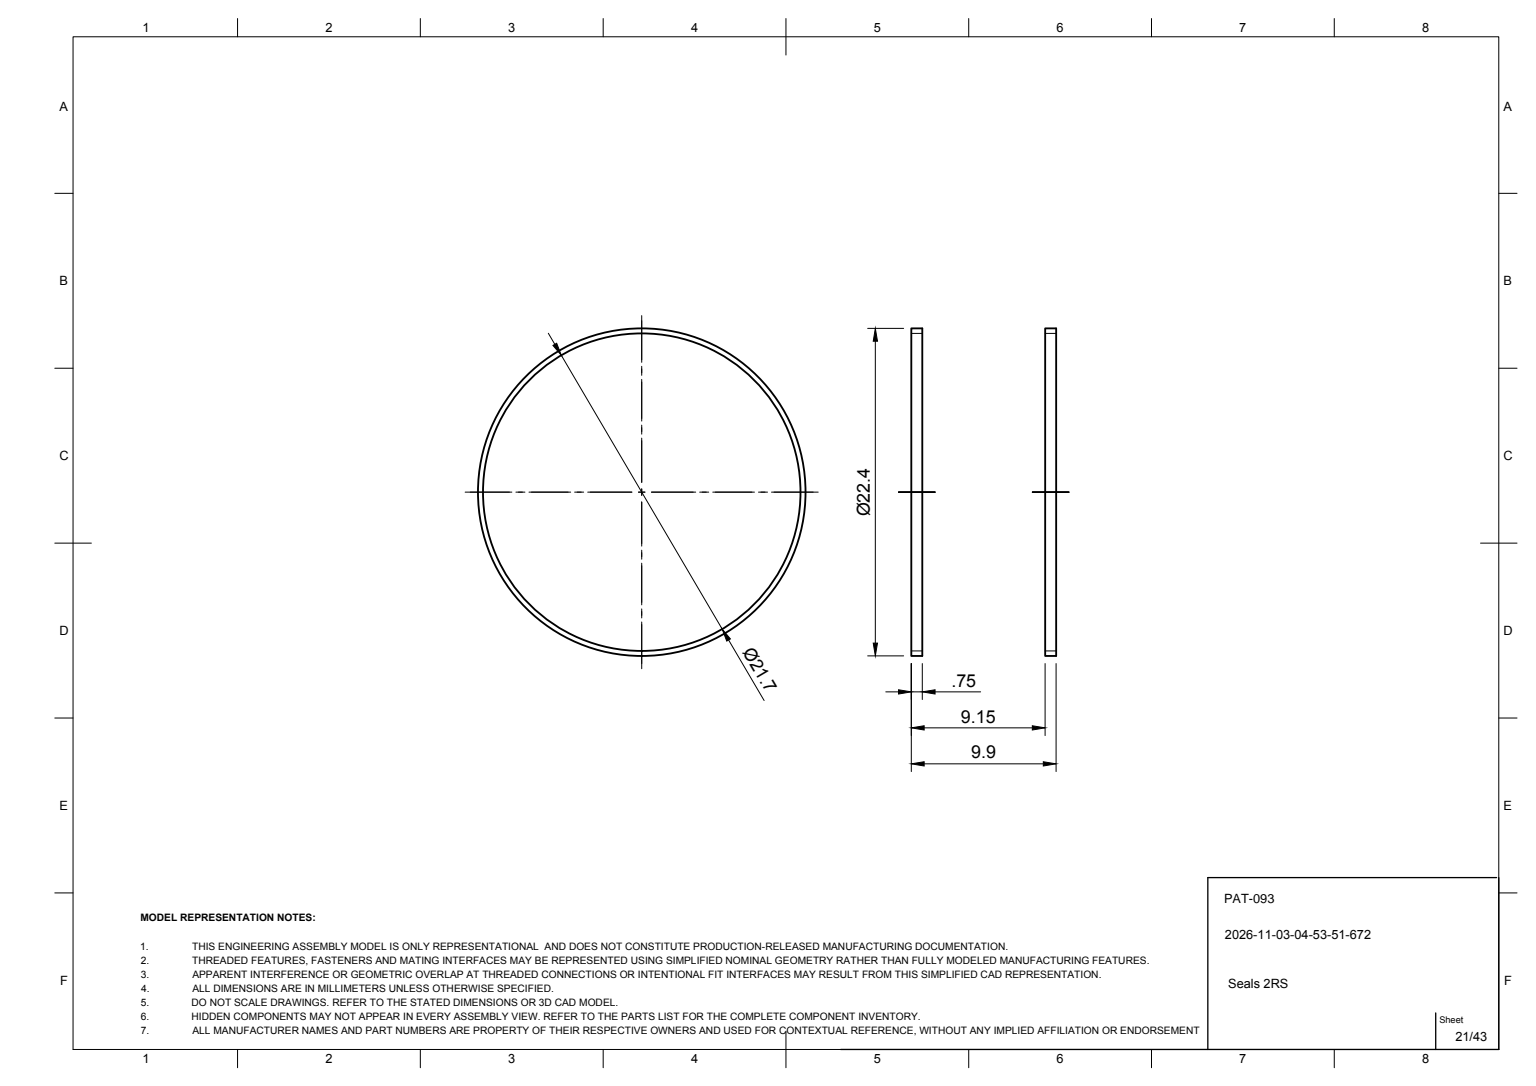
ISO-10303-21;
HEADER;
/* Generated by software containing ST-Developer
 * from STEP Tools, Inc. (www.steptools.com) 
 */

FILE_DESCRIPTION(
/* description */ ('Self-centering screw clamp'),
/* implementation_level */ '2;1');

FILE_NAME(
/* name */ 'Seals 2RS.step',
/* time_stamp */ '2026-10-28T03:25:31-07:00',
/* author */ (''),
/* organization */ (''),
/* preprocessor_version */ 'ST-DEVELOPER v20.2',
/* originating_system */ 'Autodesk Translation Framework v15.17.0.0',
/* authorisation */ '');

FILE_SCHEMA (('AUTOMOTIVE_DESIGN { 1 0 10303 214 3 1 1 }'));
ENDSEC;

DATA;
#10=MECHANICAL_DESIGN_GEOMETRIC_PRESENTATION_REPRESENTATION('',(#648,#649),#16799);
#560=SHAPE_REPRESENTATION_RELATIONSHIP('SRR','None',#17034,#601);
#601=ADVANCED_BREP_SHAPE_REPRESENTATION('',(#696,#697),#16772);
#648=STYLED_ITEM('',(#17326),#696);
#649=STYLED_ITEM('',(#17326),#697);
#696=MANIFOLD_SOLID_BREP('Body1',#9099);
#697=MANIFOLD_SOLID_BREP('Body2',#9100);
#847=FACE_BOUND('',#2128,.T.);
#848=FACE_BOUND('',#2131,.T.);
#849=FACE_BOUND('',#2134,.T.);
#850=FACE_BOUND('',#2137,.T.);
#1118=PLANE('',#10061);
#1119=PLANE('',#10066);
#1120=PLANE('',#10069);
#1121=PLANE('',#10074);
#1494=FACE_OUTER_BOUND('',#2127,.T.);
#1495=FACE_OUTER_BOUND('',#2129,.T.);
#1496=FACE_OUTER_BOUND('',#2130,.T.);
#1497=FACE_OUTER_BOUND('',#2132,.T.);
#1498=FACE_OUTER_BOUND('',#2133,.T.);
#1499=FACE_OUTER_BOUND('',#2135,.T.);
#1500=FACE_OUTER_BOUND('',#2136,.T.);
#1501=FACE_OUTER_BOUND('',#2138,.T.);
#2127=EDGE_LOOP('',(#7167));
#2128=EDGE_LOOP('',(#7168));
#2129=EDGE_LOOP('',(#7169,#7170,#7171,#7172));
#2130=EDGE_LOOP('',(#7173));
#2131=EDGE_LOOP('',(#7174));
#2132=EDGE_LOOP('',(#7175,#7176,#7177,#7178));
#2133=EDGE_LOOP('',(#7179));
#2134=EDGE_LOOP('',(#7180));
#2135=EDGE_LOOP('',(#7181,#7182,#7183,#7184));
#2136=EDGE_LOOP('',(#7185));
#2137=EDGE_LOOP('',(#7186));
#2138=EDGE_LOOP('',(#7187,#7188,#7189,#7190));
#2838=LINE('',#15182,#3411);
#2839=LINE('',#15187,#3412);
#2840=LINE('',#15196,#3413);
#2841=LINE('',#15201,#3414);
#3411=VECTOR('',#11991,1.119765);
#3412=VECTOR('',#11998,1.085235);
#3413=VECTOR('',#12009,1.119765);
#3414=VECTOR('',#12016,1.085235);
#3964=CIRCLE('',#10062,1.119765);
#3965=CIRCLE('',#10063,1.085235);
#3966=CIRCLE('',#10065,1.119765);
#3967=CIRCLE('',#10067,1.085235);
#3968=CIRCLE('',#10070,1.119765);
#3969=CIRCLE('',#10071,1.085235);
#3970=CIRCLE('',#10073,1.119765);
#3971=CIRCLE('',#10075,1.085235);
#4583=VERTEX_POINT('',#15175);
#4584=VERTEX_POINT('',#15177);
#4585=VERTEX_POINT('',#15180);
#4586=VERTEX_POINT('',#15184);
#4587=VERTEX_POINT('',#15189);
#4588=VERTEX_POINT('',#15191);
#4589=VERTEX_POINT('',#15194);
#4590=VERTEX_POINT('',#15198);
#5508=EDGE_CURVE('',#4583,#4583,#3964,.T.);
#5509=EDGE_CURVE('',#4584,#4584,#3965,.T.);
#5510=EDGE_CURVE('',#4585,#4585,#3966,.T.);
#5511=EDGE_CURVE('',#4585,#4583,#2838,.T.);
#5512=EDGE_CURVE('',#4586,#4586,#3967,.T.);
#5513=EDGE_CURVE('',#4586,#4584,#2839,.T.);
#5514=EDGE_CURVE('',#4587,#4587,#3968,.T.);
#5515=EDGE_CURVE('',#4588,#4588,#3969,.T.);
#5516=EDGE_CURVE('',#4589,#4589,#3970,.T.);
#5517=EDGE_CURVE('',#4589,#4587,#2840,.T.);
#5518=EDGE_CURVE('',#4590,#4590,#3971,.T.);
#5519=EDGE_CURVE('',#4590,#4588,#2841,.T.);
#7167=ORIENTED_EDGE('',*,*,#5508,.F.);
#7168=ORIENTED_EDGE('',*,*,#5509,.T.);
#7169=ORIENTED_EDGE('',*,*,#5510,.F.);
#7170=ORIENTED_EDGE('',*,*,#5511,.T.);
#7171=ORIENTED_EDGE('',*,*,#5508,.T.);
#7172=ORIENTED_EDGE('',*,*,#5511,.F.);
#7173=ORIENTED_EDGE('',*,*,#5510,.T.);
#7174=ORIENTED_EDGE('',*,*,#5512,.F.);
#7175=ORIENTED_EDGE('',*,*,#5512,.T.);
#7176=ORIENTED_EDGE('',*,*,#5513,.T.);
#7177=ORIENTED_EDGE('',*,*,#5509,.F.);
#7178=ORIENTED_EDGE('',*,*,#5513,.F.);
#7179=ORIENTED_EDGE('',*,*,#5514,.F.);
#7180=ORIENTED_EDGE('',*,*,#5515,.T.);
#7181=ORIENTED_EDGE('',*,*,#5516,.F.);
#7182=ORIENTED_EDGE('',*,*,#5517,.T.);
#7183=ORIENTED_EDGE('',*,*,#5514,.T.);
#7184=ORIENTED_EDGE('',*,*,#5517,.F.);
#7185=ORIENTED_EDGE('',*,*,#5516,.T.);
#7186=ORIENTED_EDGE('',*,*,#5518,.F.);
#7187=ORIENTED_EDGE('',*,*,#5518,.T.);
#7188=ORIENTED_EDGE('',*,*,#5519,.T.);
#7189=ORIENTED_EDGE('',*,*,#5515,.F.);
#7190=ORIENTED_EDGE('',*,*,#5519,.F.);
#8452=CYLINDRICAL_SURFACE('',#10064,1.119765);
#8453=CYLINDRICAL_SURFACE('',#10068,1.085235);
#8454=CYLINDRICAL_SURFACE('',#10072,1.119765);
#8455=CYLINDRICAL_SURFACE('',#10076,1.085235);
#8792=ADVANCED_FACE('',(#1494,#847),#1118,.T.);
#8793=ADVANCED_FACE('',(#1495),#8452,.T.);
#8794=ADVANCED_FACE('',(#1496,#848),#1119,.T.);
#8795=ADVANCED_FACE('',(#1497),#8453,.F.);
#8796=ADVANCED_FACE('',(#1498,#849),#1120,.T.);
#8797=ADVANCED_FACE('',(#1499),#8454,.T.);
#8798=ADVANCED_FACE('',(#1500,#850),#1121,.T.);
#8799=ADVANCED_FACE('',(#1501),#8455,.F.);
#9099=CLOSED_SHELL('',(#8792,#8793,#8794,#8795));
#9100=CLOSED_SHELL('',(#8796,#8797,#8798,#8799));
#10060=AXIS2_PLACEMENT_3D('',#15173,#11979,#11980);
#10061=AXIS2_PLACEMENT_3D('',#15174,#11981,#11982);
#10062=AXIS2_PLACEMENT_3D('',#15176,#11983,#11984);
#10063=AXIS2_PLACEMENT_3D('',#15178,#11985,#11986);
#10064=AXIS2_PLACEMENT_3D('',#15179,#11987,#11988);
#10065=AXIS2_PLACEMENT_3D('',#15181,#11989,#11990);
#10066=AXIS2_PLACEMENT_3D('',#15183,#11992,#11993);
#10067=AXIS2_PLACEMENT_3D('',#15185,#11994,#11995);
#10068=AXIS2_PLACEMENT_3D('',#15186,#11996,#11997);
#10069=AXIS2_PLACEMENT_3D('',#15188,#11999,#12000);
#10070=AXIS2_PLACEMENT_3D('',#15190,#12001,#12002);
#10071=AXIS2_PLACEMENT_3D('',#15192,#12003,#12004);
#10072=AXIS2_PLACEMENT_3D('',#15193,#12005,#12006);
#10073=AXIS2_PLACEMENT_3D('',#15195,#12007,#12008);
#10074=AXIS2_PLACEMENT_3D('',#15197,#12010,#12011);
#10075=AXIS2_PLACEMENT_3D('',#15199,#12012,#12013);
#10076=AXIS2_PLACEMENT_3D('',#15200,#12014,#12015);
#11979=DIRECTION('axis',(0.,0.,1.));
#11980=DIRECTION('refdir',(1.,0.,0.));
#11981=DIRECTION('center_axis',(0.,1.,0.));
#11982=DIRECTION('ref_axis',(0.,0.,1.));
#11983=DIRECTION('center_axis',(0.,-1.,0.));
#11984=DIRECTION('ref_axis',(1.,0.,0.));
#11985=DIRECTION('center_axis',(0.,-1.,0.));
#11986=DIRECTION('ref_axis',(1.,0.,0.));
#11987=DIRECTION('center_axis',(0.,-1.,0.));
#11988=DIRECTION('ref_axis',(1.,0.,0.));
#11989=DIRECTION('center_axis',(0.,-1.,0.));
#11990=DIRECTION('ref_axis',(1.,0.,0.));
#11991=DIRECTION('',(0.,1.,0.));
#11992=DIRECTION('center_axis',(0.,-1.,0.));
#11993=DIRECTION('ref_axis',(0.,0.,-1.));
#11994=DIRECTION('center_axis',(0.,-1.,0.));
#11995=DIRECTION('ref_axis',(1.,0.,0.));
#11996=DIRECTION('center_axis',(0.,-1.,0.));
#11997=DIRECTION('ref_axis',(1.,0.,0.));
#11998=DIRECTION('',(0.,1.,0.));
#11999=DIRECTION('center_axis',(0.,1.,0.));
#12000=DIRECTION('ref_axis',(0.,0.,1.));
#12001=DIRECTION('center_axis',(0.,-1.,0.));
#12002=DIRECTION('ref_axis',(1.,0.,0.));
#12003=DIRECTION('center_axis',(0.,-1.,0.));
#12004=DIRECTION('ref_axis',(1.,0.,0.));
#12005=DIRECTION('center_axis',(0.,-1.,0.));
#12006=DIRECTION('ref_axis',(1.,0.,0.));
#12007=DIRECTION('center_axis',(0.,-1.,0.));
#12008=DIRECTION('ref_axis',(1.,0.,0.));
#12009=DIRECTION('',(0.,1.,0.));
#12010=DIRECTION('center_axis',(0.,-1.,0.));
#12011=DIRECTION('ref_axis',(0.,0.,-1.));
#12012=DIRECTION('center_axis',(0.,-1.,0.));
#12013=DIRECTION('ref_axis',(1.,0.,0.));
#12014=DIRECTION('center_axis',(0.,-1.,0.));
#12015=DIRECTION('ref_axis',(1.,0.,0.));
#12016=DIRECTION('',(0.,1.,0.));
#15173=CARTESIAN_POINT('',(0.,0.,0.));
#15174=CARTESIAN_POINT('Origin',(1.119765,0.495,0.));
#15175=CARTESIAN_POINT('',(-1.119765,0.495,-1.37131662304724E-16));
#15176=CARTESIAN_POINT('Origin',(0.,0.495,0.));
#15177=CARTESIAN_POINT('',(-1.085235,0.495,-1.32902956907268E-16));
#15178=CARTESIAN_POINT('Origin',(0.,0.495,0.));
#15179=CARTESIAN_POINT('Origin',(0.,0.4575,0.));
#15180=CARTESIAN_POINT('',(-1.119765,0.42,-1.37131662304724E-16));
#15181=CARTESIAN_POINT('Origin',(0.,0.42,0.));
#15182=CARTESIAN_POINT('',(-1.119765,0.4575,-1.37131662304724E-16));
#15183=CARTESIAN_POINT('Origin',(1.085235,0.42,0.));
#15184=CARTESIAN_POINT('',(-1.085235,0.42,-1.32902956907268E-16));
#15185=CARTESIAN_POINT('Origin',(0.,0.42,0.));
#15186=CARTESIAN_POINT('Origin',(0.,0.4575,0.));
#15187=CARTESIAN_POINT('',(-1.085235,0.4575,-1.32902956907268E-16));
#15188=CARTESIAN_POINT('Origin',(1.119765,-0.42,0.));
#15189=CARTESIAN_POINT('',(-1.119765,-0.42,-1.37131662304724E-16));
#15190=CARTESIAN_POINT('Origin',(0.,-0.42,0.));
#15191=CARTESIAN_POINT('',(-1.085235,-0.42,-1.32902956907268E-16));
#15192=CARTESIAN_POINT('Origin',(0.,-0.42,0.));
#15193=CARTESIAN_POINT('Origin',(0.,-0.4575,0.));
#15194=CARTESIAN_POINT('',(-1.119765,-0.495,-1.37131662304724E-16));
#15195=CARTESIAN_POINT('Origin',(0.,-0.495,0.));
#15196=CARTESIAN_POINT('',(-1.119765,-0.4575,-1.37131662304724E-16));
#15197=CARTESIAN_POINT('Origin',(1.085235,-0.495,0.));
#15198=CARTESIAN_POINT('',(-1.085235,-0.495,-1.32902956907268E-16));
#15199=CARTESIAN_POINT('Origin',(0.,-0.495,0.));
#15200=CARTESIAN_POINT('Origin',(0.,-0.4575,0.));
#15201=CARTESIAN_POINT('',(-1.085235,-0.4575,-1.32902956907268E-16));
#16723=UNCERTAINTY_MEASURE_WITH_UNIT(LENGTH_MEASURE(0.001),#16800,
'DISTANCE_ACCURACY_VALUE',
'Maximum model space distance between geometric entities at asserted c
onnectivities');
#16750=UNCERTAINTY_MEASURE_WITH_UNIT(LENGTH_MEASURE(0.001),#16800,
'DISTANCE_ACCURACY_VALUE',
'Maximum model space distance between geometric entities at asserted c
onnectivities');
#16772=(
GEOMETRIC_REPRESENTATION_CONTEXT(3)
GLOBAL_UNCERTAINTY_ASSIGNED_CONTEXT((#16723))
GLOBAL_UNIT_ASSIGNED_CONTEXT((#16800,#16802,#16803))
REPRESENTATION_CONTEXT('','3D')
);
#16799=(
GEOMETRIC_REPRESENTATION_CONTEXT(3)
GLOBAL_UNCERTAINTY_ASSIGNED_CONTEXT((#16750))
GLOBAL_UNIT_ASSIGNED_CONTEXT((#16800,#16802,#16803))
REPRESENTATION_CONTEXT('','3D')
);
#16800=(
LENGTH_UNIT()
NAMED_UNIT(*)
SI_UNIT(.CENTI.,.METRE.)
);
#16802=(
NAMED_UNIT(*)
PLANE_ANGLE_UNIT()
SI_UNIT($,.RADIAN.)
);
#16803=(
NAMED_UNIT(*)
SI_UNIT($,.STERADIAN.)
SOLID_ANGLE_UNIT()
);
#16825=SHAPE_DEFINITION_REPRESENTATION(#16873,#17034);
#16873=PRODUCT_DEFINITION_SHAPE('',$,#17083);
#17034=SHAPE_REPRESENTATION('',(#10060),#16772);
#17061=PRODUCT_DEFINITION_CONTEXT('part definition',#17207,'design');
#17083=PRODUCT_DEFINITION('Seals 2RS','Seals 2RS',#17131,#17061);
#17131=PRODUCT_DEFINITION_FORMATION('',$,#17230);
#17207=APPLICATION_CONTEXT(
'Core Data for Automotive Mechanical Design Process');
#17208=PRODUCT_CONTEXT('part definition',#17207,'mechanical');
#17230=PRODUCT('Seals 2RS','Seals 2RS','Seals 2RS',(#17208));
#17320=COLOUR_RGB('Grey',0.48,0.52,0.57);
#17321=FILL_AREA_STYLE_COLOUR('',#17320);
#17322=FILL_AREA_STYLE('',(#17321));
#17323=SURFACE_STYLE_FILL_AREA(#17322);
#17324=SURFACE_SIDE_STYLE('',(#17323));
#17325=SURFACE_STYLE_USAGE(.BOTH.,#17324);
#17326=PRESENTATION_STYLE_ASSIGNMENT((#17325));
ENDSEC;
END-ISO-10303-21;
